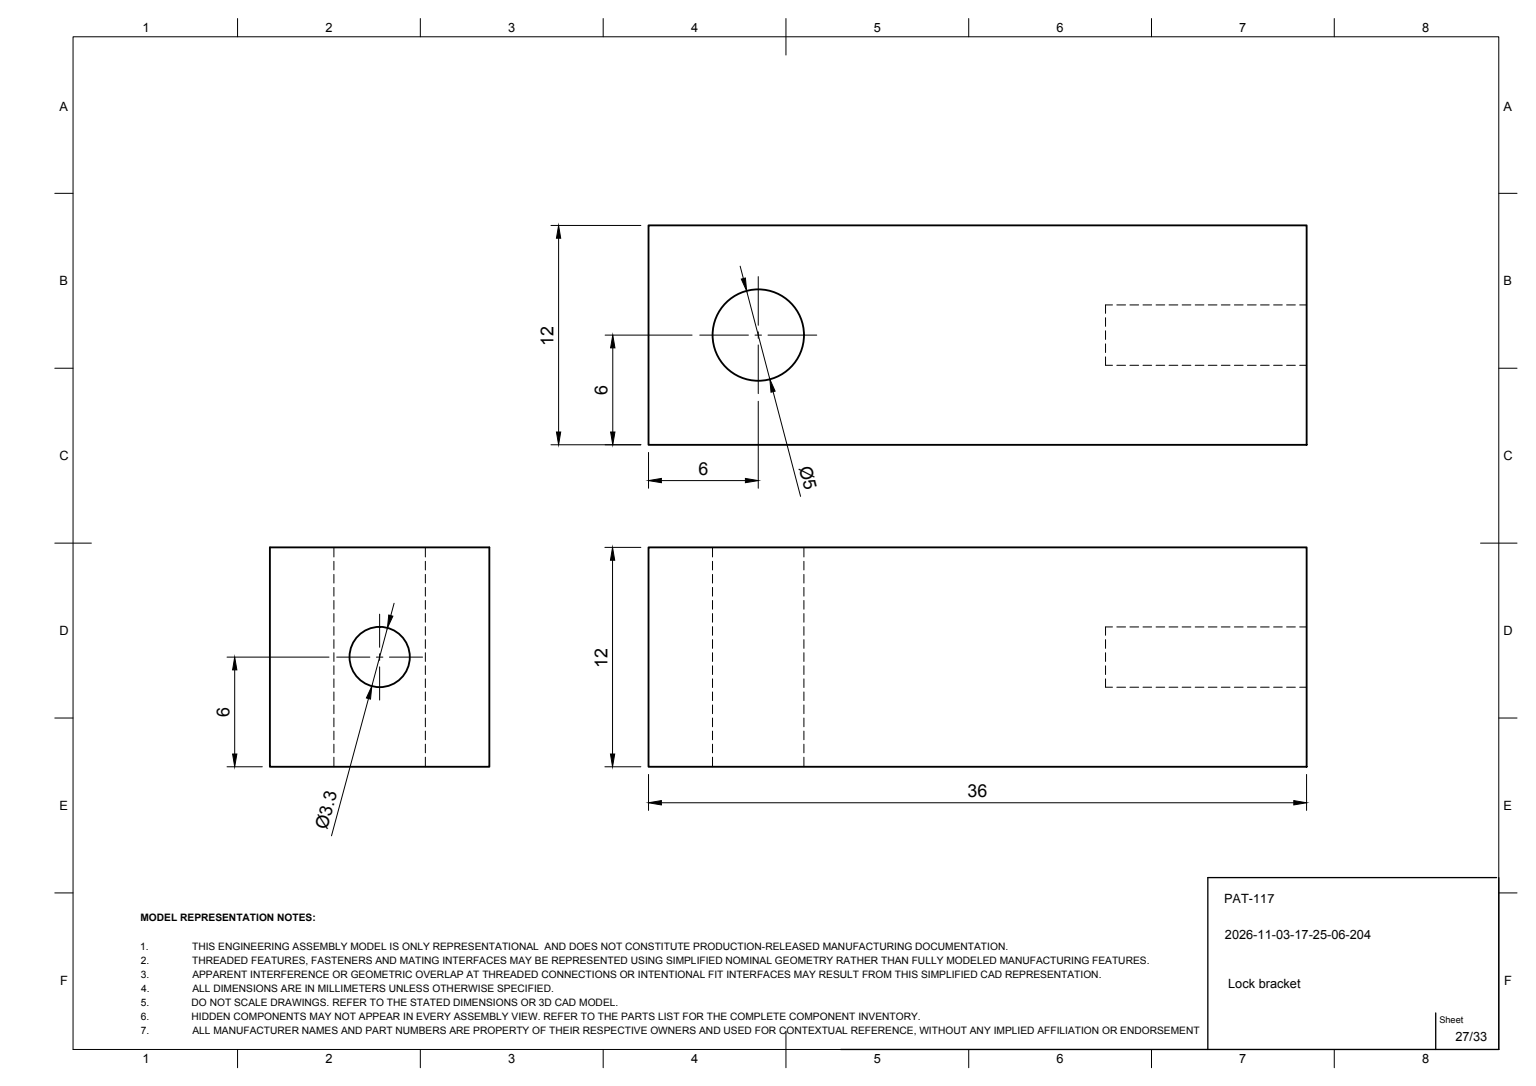
ISO-10303-21;
HEADER;
/* Generated by software containing ST-Developer
 * from STEP Tools, Inc. (www.steptools.com) 
 */

FILE_DESCRIPTION(
/* description */ ('Counterbalanced vertical column'),
/* implementation_level */ '2;1');

FILE_NAME(
/* name */ 'Lock bracket.step',
/* time_stamp */ '2026-10-29T16:47:22-07:00',
/* author */ (''),
/* organization */ (''),
/* preprocessor_version */ 'ST-DEVELOPER v20.2',
/* originating_system */ 'Autodesk Translation Framework v15.17.0.0',
/* authorisation */ '');

FILE_SCHEMA (('AUTOMOTIVE_DESIGN { 1 0 10303 214 3 1 1 }'));
ENDSEC;

DATA;
#10=MECHANICAL_DESIGN_GEOMETRIC_PRESENTATION_REPRESENTATION('',(#377),#15040);
#307=SHAPE_REPRESENTATION_RELATIONSHIP('SRR','None',#15212,#342);
#342=ADVANCED_BREP_SHAPE_REPRESENTATION('',(#410),#15031);
#377=STYLED_ITEM('',(#15436),#410);
#410=MANIFOLD_SOLID_BREP('Body1',#7102);
#521=FACE_BOUND('',#1650,.T.);
#522=FACE_BOUND('',#1653,.T.);
#523=FACE_BOUND('',#1655,.T.);
#750=PLANE('',#8026);
#751=PLANE('',#8027);
#752=PLANE('',#8028);
#753=PLANE('',#8029);
#754=PLANE('',#8030);
#755=PLANE('',#8031);
#756=PLANE('',#8032);
#1136=FACE_OUTER_BOUND('',#1646,.T.);
#1137=FACE_OUTER_BOUND('',#1647,.T.);
#1138=FACE_OUTER_BOUND('',#1648,.T.);
#1139=FACE_OUTER_BOUND('',#1649,.T.);
#1140=FACE_OUTER_BOUND('',#1651,.T.);
#1141=FACE_OUTER_BOUND('',#1652,.T.);
#1142=FACE_OUTER_BOUND('',#1654,.T.);
#1143=FACE_OUTER_BOUND('',#1656,.T.);
#1144=FACE_OUTER_BOUND('',#1657,.T.);
#1646=EDGE_LOOP('',(#6138,#6139,#6140,#6141));
#1647=EDGE_LOOP('',(#6142,#6143,#6144,#6145));
#1648=EDGE_LOOP('',(#6146));
#1649=EDGE_LOOP('',(#6147,#6148,#6149,#6150));
#1650=EDGE_LOOP('',(#6151));
#1651=EDGE_LOOP('',(#6152,#6153,#6154,#6155));
#1652=EDGE_LOOP('',(#6156,#6157,#6158,#6159));
#1653=EDGE_LOOP('',(#6160));
#1654=EDGE_LOOP('',(#6161,#6162,#6163,#6164));
#1655=EDGE_LOOP('',(#6165));
#1656=EDGE_LOOP('',(#6166,#6167,#6168,#6169));
#1657=EDGE_LOOP('',(#6170,#6171,#6172,#6173));
#2243=LINE('',#14442,#2914);
#2244=LINE('',#14448,#2915);
#2245=LINE('',#14454,#2916);
#2246=LINE('',#14456,#2917);
#2247=LINE('',#14458,#2918);
#2248=LINE('',#14459,#2919);
#2249=LINE('',#14462,#2920);
#2250=LINE('',#14464,#2921);
#2251=LINE('',#14465,#2922);
#2252=LINE('',#14468,#2923);
#2253=LINE('',#14470,#2924);
#2254=LINE('',#14471,#2925);
#2255=LINE('',#14473,#2926);
#2256=LINE('',#14474,#2927);
#2914=VECTOR('',#9761,0.25);
#2915=VECTOR('',#9768,0.164999999999999);
#2916=VECTOR('',#9775,1.);
#2917=VECTOR('',#9776,1.);
#2918=VECTOR('',#9777,1.);
#2919=VECTOR('',#9778,1.);
#2920=VECTOR('',#9781,1.);
#2921=VECTOR('',#9782,1.);
#2922=VECTOR('',#9783,1.);
#2923=VECTOR('',#9786,1.);
#2924=VECTOR('',#9787,1.);
#2925=VECTOR('',#9788,1.);
#2926=VECTOR('',#9791,1.);
#2927=VECTOR('',#9792,1.);
#3267=CIRCLE('',#8021,0.25);
#3268=CIRCLE('',#8022,0.25);
#3269=CIRCLE('',#8024,0.164999999999999);
#3270=CIRCLE('',#8025,0.164999999999999);
#3752=VERTEX_POINT('',#14439);
#3753=VERTEX_POINT('',#14441);
#3754=VERTEX_POINT('',#14445);
#3755=VERTEX_POINT('',#14447);
#3756=VERTEX_POINT('',#14452);
#3757=VERTEX_POINT('',#14453);
#3758=VERTEX_POINT('',#14455);
#3759=VERTEX_POINT('',#14457);
#3760=VERTEX_POINT('',#14461);
#3761=VERTEX_POINT('',#14463);
#3762=VERTEX_POINT('',#14467);
#3763=VERTEX_POINT('',#14469);
#4570=EDGE_CURVE('',#3752,#3752,#3267,.T.);
#4571=EDGE_CURVE('',#3752,#3753,#2243,.T.);
#4572=EDGE_CURVE('',#3753,#3753,#3268,.T.);
#4573=EDGE_CURVE('',#3754,#3754,#3269,.T.);
#4574=EDGE_CURVE('',#3754,#3755,#2244,.T.);
#4575=EDGE_CURVE('',#3755,#3755,#3270,.T.);
#4576=EDGE_CURVE('',#3756,#3757,#2245,.T.);
#4577=EDGE_CURVE('',#3757,#3758,#2246,.T.);
#4578=EDGE_CURVE('',#3759,#3758,#2247,.T.);
#4579=EDGE_CURVE('',#3756,#3759,#2248,.T.);
#4580=EDGE_CURVE('',#3760,#3756,#2249,.T.);
#4581=EDGE_CURVE('',#3761,#3759,#2250,.T.);
#4582=EDGE_CURVE('',#3760,#3761,#2251,.T.);
#4583=EDGE_CURVE('',#3762,#3760,#2252,.T.);
#4584=EDGE_CURVE('',#3763,#3761,#2253,.T.);
#4585=EDGE_CURVE('',#3762,#3763,#2254,.T.);
#4586=EDGE_CURVE('',#3757,#3762,#2255,.T.);
#4587=EDGE_CURVE('',#3758,#3763,#2256,.T.);
#6138=ORIENTED_EDGE('',*,*,#4570,.F.);
#6139=ORIENTED_EDGE('',*,*,#4571,.T.);
#6140=ORIENTED_EDGE('',*,*,#4572,.F.);
#6141=ORIENTED_EDGE('',*,*,#4571,.F.);
#6142=ORIENTED_EDGE('',*,*,#4573,.F.);
#6143=ORIENTED_EDGE('',*,*,#4574,.T.);
#6144=ORIENTED_EDGE('',*,*,#4575,.T.);
#6145=ORIENTED_EDGE('',*,*,#4574,.F.);
#6146=ORIENTED_EDGE('',*,*,#4575,.F.);
#6147=ORIENTED_EDGE('',*,*,#4576,.T.);
#6148=ORIENTED_EDGE('',*,*,#4577,.T.);
#6149=ORIENTED_EDGE('',*,*,#4578,.F.);
#6150=ORIENTED_EDGE('',*,*,#4579,.F.);
#6151=ORIENTED_EDGE('',*,*,#4572,.T.);
#6152=ORIENTED_EDGE('',*,*,#4580,.T.);
#6153=ORIENTED_EDGE('',*,*,#4579,.T.);
#6154=ORIENTED_EDGE('',*,*,#4581,.F.);
#6155=ORIENTED_EDGE('',*,*,#4582,.F.);
#6156=ORIENTED_EDGE('',*,*,#4583,.T.);
#6157=ORIENTED_EDGE('',*,*,#4582,.T.);
#6158=ORIENTED_EDGE('',*,*,#4584,.F.);
#6159=ORIENTED_EDGE('',*,*,#4585,.F.);
#6160=ORIENTED_EDGE('',*,*,#4570,.T.);
#6161=ORIENTED_EDGE('',*,*,#4586,.T.);
#6162=ORIENTED_EDGE('',*,*,#4585,.T.);
#6163=ORIENTED_EDGE('',*,*,#4587,.F.);
#6164=ORIENTED_EDGE('',*,*,#4577,.F.);
#6165=ORIENTED_EDGE('',*,*,#4573,.T.);
#6166=ORIENTED_EDGE('',*,*,#4587,.T.);
#6167=ORIENTED_EDGE('',*,*,#4584,.T.);
#6168=ORIENTED_EDGE('',*,*,#4581,.T.);
#6169=ORIENTED_EDGE('',*,*,#4578,.T.);
#6170=ORIENTED_EDGE('',*,*,#4586,.F.);
#6171=ORIENTED_EDGE('',*,*,#4576,.F.);
#6172=ORIENTED_EDGE('',*,*,#4580,.F.);
#6173=ORIENTED_EDGE('',*,*,#4583,.F.);
#6656=CYLINDRICAL_SURFACE('',#8020,0.25);
#6657=CYLINDRICAL_SURFACE('',#8023,0.164999999999999);
#6978=ADVANCED_FACE('',(#1136),#6656,.F.);
#6979=ADVANCED_FACE('',(#1137),#6657,.F.);
#6980=ADVANCED_FACE('',(#1138),#750,.F.);
#6981=ADVANCED_FACE('',(#1139,#521),#751,.T.);
#6982=ADVANCED_FACE('',(#1140),#752,.T.);
#6983=ADVANCED_FACE('',(#1141,#522),#753,.T.);
#6984=ADVANCED_FACE('',(#1142,#523),#754,.T.);
#6985=ADVANCED_FACE('',(#1143),#755,.T.);
#6986=ADVANCED_FACE('',(#1144),#756,.F.);
#7102=CLOSED_SHELL('',(#6978,#6979,#6980,#6981,#6982,#6983,#6984,#6985,
#6986));
#8019=AXIS2_PLACEMENT_3D('',#14437,#9755,#9756);
#8020=AXIS2_PLACEMENT_3D('',#14438,#9757,#9758);
#8021=AXIS2_PLACEMENT_3D('',#14440,#9759,#9760);
#8022=AXIS2_PLACEMENT_3D('',#14443,#9762,#9763);
#8023=AXIS2_PLACEMENT_3D('',#14444,#9764,#9765);
#8024=AXIS2_PLACEMENT_3D('',#14446,#9766,#9767);
#8025=AXIS2_PLACEMENT_3D('',#14449,#9769,#9770);
#8026=AXIS2_PLACEMENT_3D('',#14450,#9771,#9772);
#8027=AXIS2_PLACEMENT_3D('',#14451,#9773,#9774);
#8028=AXIS2_PLACEMENT_3D('',#14460,#9779,#9780);
#8029=AXIS2_PLACEMENT_3D('',#14466,#9784,#9785);
#8030=AXIS2_PLACEMENT_3D('',#14472,#9789,#9790);
#8031=AXIS2_PLACEMENT_3D('',#14475,#9793,#9794);
#8032=AXIS2_PLACEMENT_3D('',#14476,#9795,#9796);
#9755=DIRECTION('axis',(0.,0.,1.));
#9756=DIRECTION('refdir',(1.,0.,0.));
#9757=DIRECTION('center_axis',(0.,1.,0.));
#9758=DIRECTION('ref_axis',(1.,0.,0.));
#9759=DIRECTION('center_axis',(0.,1.,0.));
#9760=DIRECTION('ref_axis',(1.,0.,0.));
#9761=DIRECTION('',(0.,1.,0.));
#9762=DIRECTION('center_axis',(0.,-1.,0.));
#9763=DIRECTION('ref_axis',(1.,0.,0.));
#9764=DIRECTION('center_axis',(1.,0.,0.));
#9765=DIRECTION('ref_axis',(0.,0.,-1.));
#9766=DIRECTION('center_axis',(1.,0.,0.));
#9767=DIRECTION('ref_axis',(0.,0.,-1.));
#9768=DIRECTION('',(1.,0.,0.));
#9769=DIRECTION('center_axis',(1.,0.,0.));
#9770=DIRECTION('ref_axis',(0.,0.,-1.));
#9771=DIRECTION('center_axis',(1.,0.,0.));
#9772=DIRECTION('ref_axis',(0.,0.,-1.));
#9773=DIRECTION('center_axis',(0.,1.,0.));
#9774=DIRECTION('ref_axis',(-1.,0.,0.));
#9775=DIRECTION('',(-1.,0.,0.));
#9776=DIRECTION('',(0.,0.,1.));
#9777=DIRECTION('',(-1.,0.,0.));
#9778=DIRECTION('',(0.,0.,1.));
#9779=DIRECTION('center_axis',(1.,0.,0.));
#9780=DIRECTION('ref_axis',(0.,1.,0.));
#9781=DIRECTION('',(0.,1.,0.));
#9782=DIRECTION('',(0.,1.,0.));
#9783=DIRECTION('',(0.,0.,1.));
#9784=DIRECTION('center_axis',(0.,-1.,0.));
#9785=DIRECTION('ref_axis',(1.,0.,0.));
#9786=DIRECTION('',(1.,0.,0.));
#9787=DIRECTION('',(1.,0.,0.));
#9788=DIRECTION('',(0.,0.,1.));
#9789=DIRECTION('center_axis',(-1.,0.,0.));
#9790=DIRECTION('ref_axis',(0.,-1.,0.));
#9791=DIRECTION('',(0.,-1.,0.));
#9792=DIRECTION('',(0.,-1.,0.));
#9793=DIRECTION('center_axis',(0.,0.,1.));
#9794=DIRECTION('ref_axis',(1.,0.,0.));
#9795=DIRECTION('center_axis',(0.,0.,1.));
#9796=DIRECTION('ref_axis',(1.,0.,0.));
#14437=CARTESIAN_POINT('',(0.,0.,0.));
#14438=CARTESIAN_POINT('Origin',(1.8,-0.1,17.6));
#14439=CARTESIAN_POINT('',(1.55,2.4,17.6));
#14440=CARTESIAN_POINT('Origin',(1.8,2.4,17.6));
#14441=CARTESIAN_POINT('',(1.55,3.6,17.6));
#14442=CARTESIAN_POINT('',(1.55,-0.1,17.6));
#14443=CARTESIAN_POINT('Origin',(1.8,3.6,17.6));
#14444=CARTESIAN_POINT('Origin',(-1.3,3.,17.6));
#14445=CARTESIAN_POINT('',(-1.2,3.,17.765));
#14446=CARTESIAN_POINT('Origin',(-1.2,3.,17.6));
#14447=CARTESIAN_POINT('',(-0.0999999999999999,3.,17.765));
#14448=CARTESIAN_POINT('',(-1.3,3.,17.765));
#14449=CARTESIAN_POINT('Origin',(-0.0999999999999999,3.,17.6));
#14450=CARTESIAN_POINT('Origin',(-0.0999999999999999,3.,17.6));
#14451=CARTESIAN_POINT('Origin',(2.4,3.6,17.));
#14452=CARTESIAN_POINT('',(2.4,3.6,17.));
#14453=CARTESIAN_POINT('',(-1.2,3.6,17.));
#14454=CARTESIAN_POINT('',(2.4,3.6,17.));
#14455=CARTESIAN_POINT('',(-1.2,3.6,18.2));
#14456=CARTESIAN_POINT('',(-1.2,3.6,17.));
#14457=CARTESIAN_POINT('',(2.4,3.6,18.2));
#14458=CARTESIAN_POINT('',(2.4,3.6,18.2));
#14459=CARTESIAN_POINT('',(2.4,3.6,17.));
#14460=CARTESIAN_POINT('Origin',(2.4,2.4,17.));
#14461=CARTESIAN_POINT('',(2.4,2.4,17.));
#14462=CARTESIAN_POINT('',(2.4,2.4,17.));
#14463=CARTESIAN_POINT('',(2.4,2.4,18.2));
#14464=CARTESIAN_POINT('',(2.4,2.4,18.2));
#14465=CARTESIAN_POINT('',(2.4,2.4,17.));
#14466=CARTESIAN_POINT('Origin',(-1.2,2.4,17.));
#14467=CARTESIAN_POINT('',(-1.2,2.4,17.));
#14468=CARTESIAN_POINT('',(-1.2,2.4,17.));
#14469=CARTESIAN_POINT('',(-1.2,2.4,18.2));
#14470=CARTESIAN_POINT('',(-1.2,2.4,18.2));
#14471=CARTESIAN_POINT('',(-1.2,2.4,17.));
#14472=CARTESIAN_POINT('Origin',(-1.2,3.6,17.));
#14473=CARTESIAN_POINT('',(-1.2,3.6,17.));
#14474=CARTESIAN_POINT('',(-1.2,3.6,18.2));
#14475=CARTESIAN_POINT('Origin',(0.6,3.,18.2));
#14476=CARTESIAN_POINT('Origin',(0.6,3.,17.));
#14991=UNCERTAINTY_MEASURE_WITH_UNIT(LENGTH_MEASURE(0.001),#15041,
'DISTANCE_ACCURACY_VALUE',
'Maximum model space distance between geometric entities at asserted c
onnectivities');
#15000=UNCERTAINTY_MEASURE_WITH_UNIT(LENGTH_MEASURE(0.001),#15041,
'DISTANCE_ACCURACY_VALUE',
'Maximum model space distance between geometric entities at asserted c
onnectivities');
#15031=(
GEOMETRIC_REPRESENTATION_CONTEXT(3)
GLOBAL_UNCERTAINTY_ASSIGNED_CONTEXT((#14991))
GLOBAL_UNIT_ASSIGNED_CONTEXT((#15041,#15043,#15044))
REPRESENTATION_CONTEXT('','3D')
);
#15040=(
GEOMETRIC_REPRESENTATION_CONTEXT(3)
GLOBAL_UNCERTAINTY_ASSIGNED_CONTEXT((#15000))
GLOBAL_UNIT_ASSIGNED_CONTEXT((#15041,#15043,#15044))
REPRESENTATION_CONTEXT('','3D')
);
#15041=(
LENGTH_UNIT()
NAMED_UNIT(*)
SI_UNIT(.CENTI.,.METRE.)
);
#15043=(
NAMED_UNIT(*)
PLANE_ANGLE_UNIT()
SI_UNIT($,.RADIAN.)
);
#15044=(
NAMED_UNIT(*)
SI_UNIT($,.STERADIAN.)
SOLID_ANGLE_UNIT()
);
#15075=SHAPE_DEFINITION_REPRESENTATION(#15114,#15212);
#15114=PRODUCT_DEFINITION_SHAPE('',$,#15252);
#15212=SHAPE_REPRESENTATION('',(#8019),#15031);
#15221=PRODUCT_DEFINITION_CONTEXT('part definition',#15340,'design');
#15252=PRODUCT_DEFINITION('Lock bracket','Lock bracket',#15291,#15221);
#15291=PRODUCT_DEFINITION_FORMATION('',$,#15372);
#15340=APPLICATION_CONTEXT(
'Core Data for Automotive Mechanical Design Process');
#15341=PRODUCT_CONTEXT('part definition',#15340,'mechanical');
#15372=PRODUCT('Lock bracket','Lock bracket','Lock bracket',(#15341));
#15430=COLOUR_RGB('Dark Blue',0.08,0.2,0.34);
#15431=FILL_AREA_STYLE_COLOUR('',#15430);
#15432=FILL_AREA_STYLE('',(#15431));
#15433=SURFACE_STYLE_FILL_AREA(#15432);
#15434=SURFACE_SIDE_STYLE('',(#15433));
#15435=SURFACE_STYLE_USAGE(.BOTH.,#15434);
#15436=PRESENTATION_STYLE_ASSIGNMENT((#15435));
ENDSEC;
END-ISO-10303-21;
